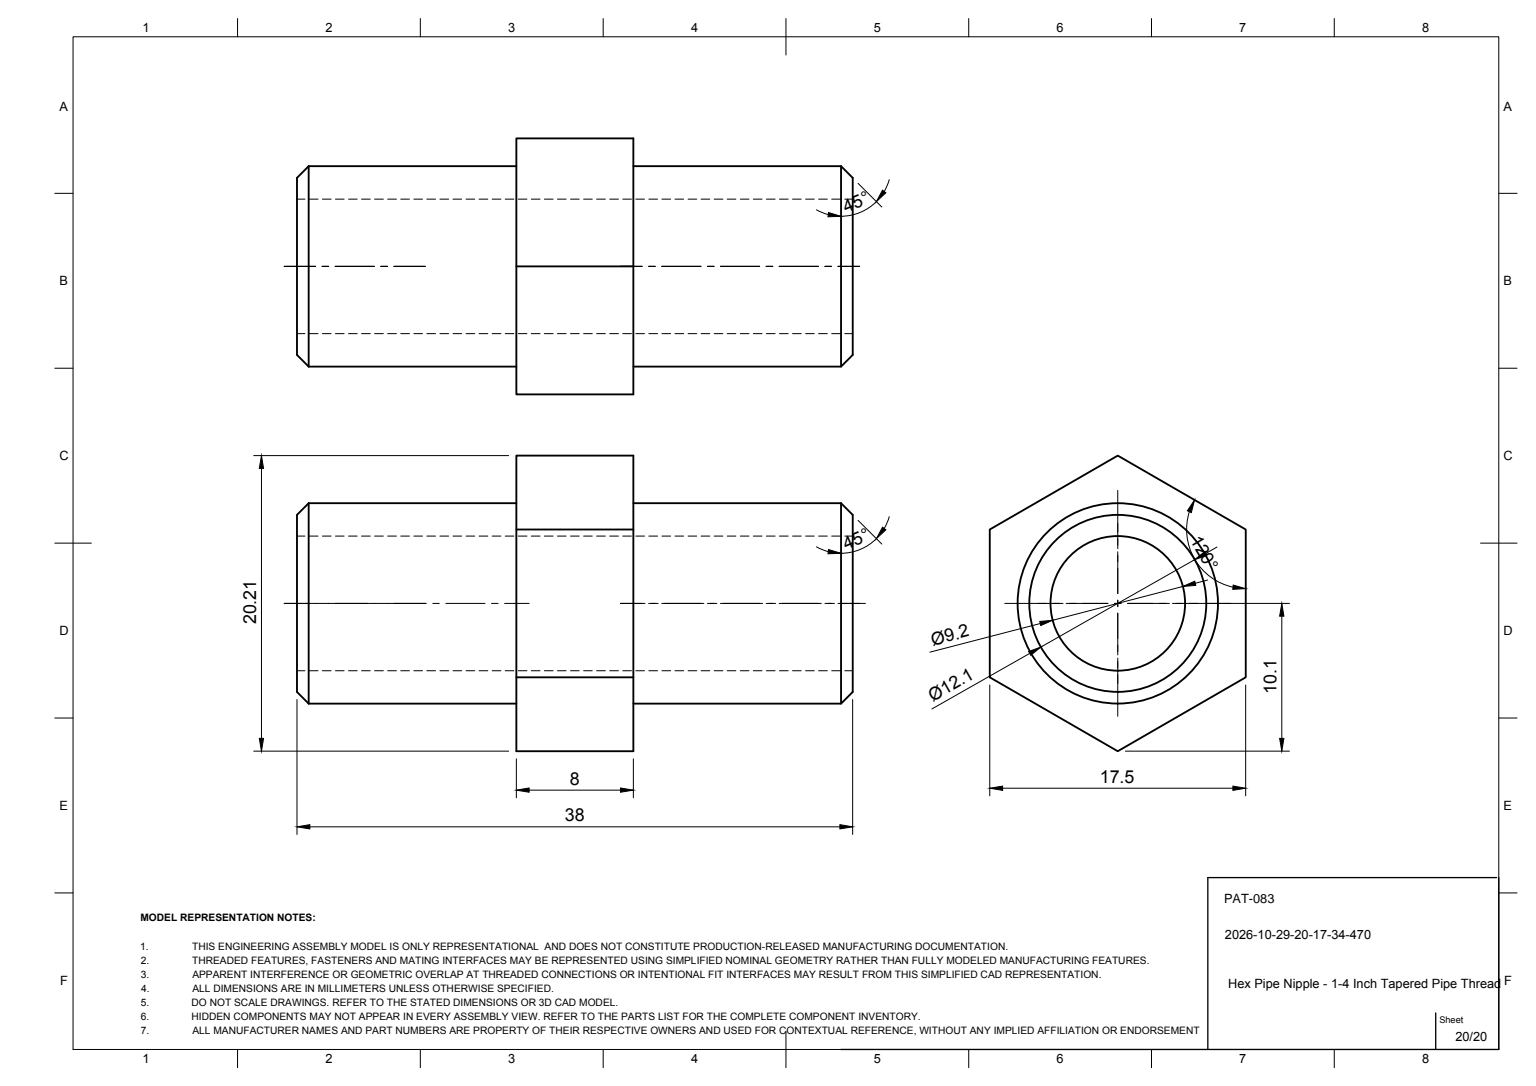
ISO-10303-21;
HEADER;
/* Generated by software containing ST-Developer
 * from STEP Tools, Inc. (www.steptools.com) 
 */

FILE_DESCRIPTION(
/* description */ ('PAT-083'),
/* implementation_level */ '2;1');

FILE_NAME(
/* name */ 'Hex Pipe Nipple - 1-4 Inch Tapered Pipe Thread.step',
/* time_stamp */ '2026-10-29T20:18:00-07:00',
/* author */ (''),
/* organization */ (''),
/* preprocessor_version */ 'ST-DEVELOPER v20.2',
/* originating_system */ 'Autodesk Translation Framework v15.17.0.0',
/* authorisation */ '');

FILE_SCHEMA (('AUTOMOTIVE_DESIGN { 1 0 10303 214 3 1 1 }'));
ENDSEC;

DATA;
#10=MECHANICAL_DESIGN_GEOMETRIC_PRESENTATION_REPRESENTATION('',(#248),#8428);
#153=CONICAL_SURFACE('',#4329,0.645,0.785398163397448);
#154=CONICAL_SURFACE('',#4332,0.645,0.785398163397448);
#200=SHAPE_REPRESENTATION_RELATIONSHIP('SRR','None',#8534,#224);
#224=ADVANCED_BREP_SHAPE_REPRESENTATION('',(#271),#8423);
#248=STYLED_ITEM('',(#8698),#271);
#271=MANIFOLD_SOLID_BREP('Body1',#3695);
#346=FACE_BOUND('',#974,.T.);
#347=FACE_BOUND('',#976,.T.);
#348=FACE_BOUND('',#985,.T.);
#349=FACE_BOUND('',#990,.T.);
#455=PLANE('',#4314);
#456=PLANE('',#4316);
#457=PLANE('',#4318);
#458=PLANE('',#4319);
#459=PLANE('',#4320);
#460=PLANE('',#4321);
#461=PLANE('',#4322);
#462=PLANE('',#4323);
#463=PLANE('',#4326);
#464=PLANE('',#4334);
#669=FACE_OUTER_BOUND('',#973,.T.);
#670=FACE_OUTER_BOUND('',#975,.T.);
#671=FACE_OUTER_BOUND('',#977,.T.);
#672=FACE_OUTER_BOUND('',#978,.T.);
#673=FACE_OUTER_BOUND('',#979,.T.);
#674=FACE_OUTER_BOUND('',#980,.T.);
#675=FACE_OUTER_BOUND('',#981,.T.);
#676=FACE_OUTER_BOUND('',#982,.T.);
#677=FACE_OUTER_BOUND('',#983,.T.);
#678=FACE_OUTER_BOUND('',#984,.T.);
#679=FACE_OUTER_BOUND('',#986,.T.);
#680=FACE_OUTER_BOUND('',#987,.T.);
#681=FACE_OUTER_BOUND('',#988,.T.);
#682=FACE_OUTER_BOUND('',#989,.T.);
#683=FACE_OUTER_BOUND('',#991,.T.);
#973=EDGE_LOOP('',(#3126,#3127,#3128,#3129,#3130,#3131));
#974=EDGE_LOOP('',(#3132));
#975=EDGE_LOOP('',(#3133,#3134,#3135,#3136,#3137,#3138));
#976=EDGE_LOOP('',(#3139));
#977=EDGE_LOOP('',(#3140,#3141,#3142,#3143));
#978=EDGE_LOOP('',(#3144,#3145,#3146,#3147));
#979=EDGE_LOOP('',(#3148,#3149,#3150,#3151));
#980=EDGE_LOOP('',(#3152,#3153,#3154,#3155));
#981=EDGE_LOOP('',(#3156,#3157,#3158,#3159));
#982=EDGE_LOOP('',(#3160,#3161,#3162,#3163));
#983=EDGE_LOOP('',(#3164,#3165,#3166,#3167));
#984=EDGE_LOOP('',(#3168));
#985=EDGE_LOOP('',(#3169));
#986=EDGE_LOOP('',(#3170,#3171,#3172,#3173));
#987=EDGE_LOOP('',(#3174,#3175,#3176,#3177));
#988=EDGE_LOOP('',(#3178,#3179,#3180,#3181));
#989=EDGE_LOOP('',(#3182));
#990=EDGE_LOOP('',(#3183));
#991=EDGE_LOOP('',(#3184,#3185,#3186,#3187));
#1207=LINE('',#8067,#1451);
#1208=LINE('',#8069,#1452);
#1209=LINE('',#8071,#1453);
#1210=LINE('',#8073,#1454);
#1211=LINE('',#8075,#1455);
#1212=LINE('',#8076,#1456);
#1213=LINE('',#8082,#1457);
#1214=LINE('',#8084,#1458);
#1215=LINE('',#8086,#1459);
#1216=LINE('',#8088,#1460);
#1217=LINE('',#8090,#1461);
#1218=LINE('',#8091,#1462);
#1219=LINE('',#8095,#1463);
#1220=LINE('',#8096,#1464);
#1221=LINE('',#8098,#1465);
#1222=LINE('',#8100,#1466);
#1223=LINE('',#8102,#1467);
#1224=LINE('',#8104,#1468);
#1225=LINE('',#8108,#1469);
#1226=LINE('',#8116,#1470);
#1227=LINE('',#8120,#1471);
#1228=LINE('',#8124,#1472);
#1229=LINE('',#8129,#1473);
#1451=VECTOR('',#5299,1.);
#1452=VECTOR('',#5300,1.);
#1453=VECTOR('',#5301,1.);
#1454=VECTOR('',#5302,1.);
#1455=VECTOR('',#5303,1.);
#1456=VECTOR('',#5304,1.);
#1457=VECTOR('',#5309,1.);
#1458=VECTOR('',#5310,1.);
#1459=VECTOR('',#5311,1.);
#1460=VECTOR('',#5312,1.);
#1461=VECTOR('',#5313,1.);
#1462=VECTOR('',#5314,1.);
#1463=VECTOR('',#5319,1.);
#1464=VECTOR('',#5320,1.);
#1465=VECTOR('',#5323,1.);
#1466=VECTOR('',#5326,1.);
#1467=VECTOR('',#5329,1.);
#1468=VECTOR('',#5332,1.);
#1469=VECTOR('',#5337,0.685);
#1470=VECTOR('',#5348,0.645);
#1471=VECTOR('',#5353,0.685);
#1472=VECTOR('',#5358,0.645);
#1473=VECTOR('',#5365,0.46);
#1685=CIRCLE('',#4315,0.685);
#1686=CIRCLE('',#4317,0.685);
#1687=CIRCLE('',#4325,0.685);
#1688=CIRCLE('',#4327,0.605);
#1689=CIRCLE('',#4328,0.46);
#1690=CIRCLE('',#4331,0.685);
#1691=CIRCLE('',#4333,0.605);
#1692=CIRCLE('',#4335,0.46);
#1929=VERTEX_POINT('',#8065);
#1930=VERTEX_POINT('',#8066);
#1931=VERTEX_POINT('',#8068);
#1932=VERTEX_POINT('',#8070);
#1933=VERTEX_POINT('',#8072);
#1934=VERTEX_POINT('',#8074);
#1935=VERTEX_POINT('',#8077);
#1936=VERTEX_POINT('',#8080);
#1937=VERTEX_POINT('',#8081);
#1938=VERTEX_POINT('',#8083);
#1939=VERTEX_POINT('',#8085);
#1940=VERTEX_POINT('',#8087);
#1941=VERTEX_POINT('',#8089);
#1942=VERTEX_POINT('',#8092);
#1943=VERTEX_POINT('',#8107);
#1944=VERTEX_POINT('',#8111);
#1945=VERTEX_POINT('',#8113);
#1946=VERTEX_POINT('',#8118);
#1947=VERTEX_POINT('',#8122);
#1948=VERTEX_POINT('',#8126);
#2339=EDGE_CURVE('',#1929,#1930,#1207,.T.);
#2340=EDGE_CURVE('',#1930,#1931,#1208,.T.);
#2341=EDGE_CURVE('',#1931,#1932,#1209,.T.);
#2342=EDGE_CURVE('',#1932,#1933,#1210,.T.);
#2343=EDGE_CURVE('',#1933,#1934,#1211,.T.);
#2344=EDGE_CURVE('',#1934,#1929,#1212,.T.);
#2345=EDGE_CURVE('',#1935,#1935,#1685,.T.);
#2346=EDGE_CURVE('',#1936,#1937,#1213,.T.);
#2347=EDGE_CURVE('',#1937,#1938,#1214,.T.);
#2348=EDGE_CURVE('',#1938,#1939,#1215,.T.);
#2349=EDGE_CURVE('',#1939,#1940,#1216,.T.);
#2350=EDGE_CURVE('',#1940,#1941,#1217,.T.);
#2351=EDGE_CURVE('',#1941,#1936,#1218,.T.);
#2352=EDGE_CURVE('',#1942,#1942,#1686,.T.);
#2353=EDGE_CURVE('',#1936,#1930,#1219,.T.);
#2354=EDGE_CURVE('',#1931,#1941,#1220,.T.);
#2355=EDGE_CURVE('',#1932,#1940,#1221,.T.);
#2356=EDGE_CURVE('',#1933,#1939,#1222,.T.);
#2357=EDGE_CURVE('',#1934,#1938,#1223,.T.);
#2358=EDGE_CURVE('',#1929,#1937,#1224,.T.);
#2359=EDGE_CURVE('',#1942,#1943,#1225,.T.);
#2360=EDGE_CURVE('',#1943,#1943,#1687,.T.);
#2361=EDGE_CURVE('',#1944,#1944,#1688,.T.);
#2362=EDGE_CURVE('',#1945,#1945,#1689,.T.);
#2363=EDGE_CURVE('',#1943,#1944,#1226,.T.);
#2364=EDGE_CURVE('',#1946,#1946,#1690,.T.);
#2365=EDGE_CURVE('',#1946,#1935,#1227,.T.);
#2366=EDGE_CURVE('',#1947,#1947,#1691,.T.);
#2367=EDGE_CURVE('',#1947,#1946,#1228,.T.);
#2368=EDGE_CURVE('',#1948,#1948,#1692,.T.);
#2369=EDGE_CURVE('',#1948,#1945,#1229,.T.);
#3126=ORIENTED_EDGE('',*,*,#2339,.T.);
#3127=ORIENTED_EDGE('',*,*,#2340,.T.);
#3128=ORIENTED_EDGE('',*,*,#2341,.T.);
#3129=ORIENTED_EDGE('',*,*,#2342,.T.);
#3130=ORIENTED_EDGE('',*,*,#2343,.T.);
#3131=ORIENTED_EDGE('',*,*,#2344,.T.);
#3132=ORIENTED_EDGE('',*,*,#2345,.F.);
#3133=ORIENTED_EDGE('',*,*,#2346,.T.);
#3134=ORIENTED_EDGE('',*,*,#2347,.T.);
#3135=ORIENTED_EDGE('',*,*,#2348,.T.);
#3136=ORIENTED_EDGE('',*,*,#2349,.T.);
#3137=ORIENTED_EDGE('',*,*,#2350,.T.);
#3138=ORIENTED_EDGE('',*,*,#2351,.T.);
#3139=ORIENTED_EDGE('',*,*,#2352,.F.);
#3140=ORIENTED_EDGE('',*,*,#2353,.F.);
#3141=ORIENTED_EDGE('',*,*,#2351,.F.);
#3142=ORIENTED_EDGE('',*,*,#2354,.F.);
#3143=ORIENTED_EDGE('',*,*,#2340,.F.);
#3144=ORIENTED_EDGE('',*,*,#2354,.T.);
#3145=ORIENTED_EDGE('',*,*,#2350,.F.);
#3146=ORIENTED_EDGE('',*,*,#2355,.F.);
#3147=ORIENTED_EDGE('',*,*,#2341,.F.);
#3148=ORIENTED_EDGE('',*,*,#2355,.T.);
#3149=ORIENTED_EDGE('',*,*,#2349,.F.);
#3150=ORIENTED_EDGE('',*,*,#2356,.F.);
#3151=ORIENTED_EDGE('',*,*,#2342,.F.);
#3152=ORIENTED_EDGE('',*,*,#2356,.T.);
#3153=ORIENTED_EDGE('',*,*,#2348,.F.);
#3154=ORIENTED_EDGE('',*,*,#2357,.F.);
#3155=ORIENTED_EDGE('',*,*,#2343,.F.);
#3156=ORIENTED_EDGE('',*,*,#2357,.T.);
#3157=ORIENTED_EDGE('',*,*,#2347,.F.);
#3158=ORIENTED_EDGE('',*,*,#2358,.F.);
#3159=ORIENTED_EDGE('',*,*,#2344,.F.);
#3160=ORIENTED_EDGE('',*,*,#2358,.T.);
#3161=ORIENTED_EDGE('',*,*,#2346,.F.);
#3162=ORIENTED_EDGE('',*,*,#2353,.T.);
#3163=ORIENTED_EDGE('',*,*,#2339,.F.);
#3164=ORIENTED_EDGE('',*,*,#2352,.T.);
#3165=ORIENTED_EDGE('',*,*,#2359,.T.);
#3166=ORIENTED_EDGE('',*,*,#2360,.T.);
#3167=ORIENTED_EDGE('',*,*,#2359,.F.);
#3168=ORIENTED_EDGE('',*,*,#2361,.F.);
#3169=ORIENTED_EDGE('',*,*,#2362,.T.);
#3170=ORIENTED_EDGE('',*,*,#2360,.F.);
#3171=ORIENTED_EDGE('',*,*,#2363,.T.);
#3172=ORIENTED_EDGE('',*,*,#2361,.T.);
#3173=ORIENTED_EDGE('',*,*,#2363,.F.);
#3174=ORIENTED_EDGE('',*,*,#2364,.F.);
#3175=ORIENTED_EDGE('',*,*,#2365,.T.);
#3176=ORIENTED_EDGE('',*,*,#2345,.T.);
#3177=ORIENTED_EDGE('',*,*,#2365,.F.);
#3178=ORIENTED_EDGE('',*,*,#2366,.F.);
#3179=ORIENTED_EDGE('',*,*,#2367,.T.);
#3180=ORIENTED_EDGE('',*,*,#2364,.T.);
#3181=ORIENTED_EDGE('',*,*,#2367,.F.);
#3182=ORIENTED_EDGE('',*,*,#2366,.T.);
#3183=ORIENTED_EDGE('',*,*,#2368,.F.);
#3184=ORIENTED_EDGE('',*,*,#2368,.T.);
#3185=ORIENTED_EDGE('',*,*,#2369,.T.);
#3186=ORIENTED_EDGE('',*,*,#2362,.F.);
#3187=ORIENTED_EDGE('',*,*,#2369,.F.);
#3433=CYLINDRICAL_SURFACE('',#4324,0.685);
#3434=CYLINDRICAL_SURFACE('',#4330,0.685);
#3435=CYLINDRICAL_SURFACE('',#4336,0.46);
#3616=ADVANCED_FACE('',(#669,#346),#455,.F.);
#3617=ADVANCED_FACE('',(#670,#347),#456,.T.);
#3618=ADVANCED_FACE('',(#671),#457,.T.);
#3619=ADVANCED_FACE('',(#672),#458,.T.);
#3620=ADVANCED_FACE('',(#673),#459,.T.);
#3621=ADVANCED_FACE('',(#674),#460,.T.);
#3622=ADVANCED_FACE('',(#675),#461,.T.);
#3623=ADVANCED_FACE('',(#676),#462,.T.);
#3624=ADVANCED_FACE('',(#677),#3433,.T.);
#3625=ADVANCED_FACE('',(#678,#348),#463,.T.);
#3626=ADVANCED_FACE('',(#679),#153,.T.);
#3627=ADVANCED_FACE('',(#680),#3434,.T.);
#3628=ADVANCED_FACE('',(#681),#154,.T.);
#3629=ADVANCED_FACE('',(#682,#349),#464,.T.);
#3630=ADVANCED_FACE('',(#683),#3435,.F.);
#3695=CLOSED_SHELL('',(#3616,#3617,#3618,#3619,#3620,#3621,#3622,#3623,
#3624,#3625,#3626,#3627,#3628,#3629,#3630));
#4313=AXIS2_PLACEMENT_3D('',#8063,#5295,#5296);
#4314=AXIS2_PLACEMENT_3D('',#8064,#5297,#5298);
#4315=AXIS2_PLACEMENT_3D('',#8078,#5305,#5306);
#4316=AXIS2_PLACEMENT_3D('',#8079,#5307,#5308);
#4317=AXIS2_PLACEMENT_3D('',#8093,#5315,#5316);
#4318=AXIS2_PLACEMENT_3D('',#8094,#5317,#5318);
#4319=AXIS2_PLACEMENT_3D('',#8097,#5321,#5322);
#4320=AXIS2_PLACEMENT_3D('',#8099,#5324,#5325);
#4321=AXIS2_PLACEMENT_3D('',#8101,#5327,#5328);
#4322=AXIS2_PLACEMENT_3D('',#8103,#5330,#5331);
#4323=AXIS2_PLACEMENT_3D('',#8105,#5333,#5334);
#4324=AXIS2_PLACEMENT_3D('',#8106,#5335,#5336);
#4325=AXIS2_PLACEMENT_3D('',#8109,#5338,#5339);
#4326=AXIS2_PLACEMENT_3D('',#8110,#5340,#5341);
#4327=AXIS2_PLACEMENT_3D('',#8112,#5342,#5343);
#4328=AXIS2_PLACEMENT_3D('',#8114,#5344,#5345);
#4329=AXIS2_PLACEMENT_3D('',#8115,#5346,#5347);
#4330=AXIS2_PLACEMENT_3D('',#8117,#5349,#5350);
#4331=AXIS2_PLACEMENT_3D('',#8119,#5351,#5352);
#4332=AXIS2_PLACEMENT_3D('',#8121,#5354,#5355);
#4333=AXIS2_PLACEMENT_3D('',#8123,#5356,#5357);
#4334=AXIS2_PLACEMENT_3D('',#8125,#5359,#5360);
#4335=AXIS2_PLACEMENT_3D('',#8127,#5361,#5362);
#4336=AXIS2_PLACEMENT_3D('',#8128,#5363,#5364);
#5295=DIRECTION('axis',(0.,0.,1.));
#5296=DIRECTION('refdir',(1.,0.,0.));
#5297=DIRECTION('center_axis',(0.,1.,0.));
#5298=DIRECTION('ref_axis',(1.,0.,0.));
#5299=DIRECTION('',(-0.5,0.,0.866025403784439));
#5300=DIRECTION('',(-1.,0.,-3.29650746237182E-16));
#5301=DIRECTION('',(-0.5,0.,-0.866025403784439));
#5302=DIRECTION('',(0.5,0.,-0.866025403784438));
#5303=DIRECTION('',(1.,0.,0.));
#5304=DIRECTION('',(0.5,0.,0.866025403784439));
#5305=DIRECTION('center_axis',(0.,-1.,0.));
#5306=DIRECTION('ref_axis',(1.,0.,0.));
#5307=DIRECTION('center_axis',(0.,1.,0.));
#5308=DIRECTION('ref_axis',(1.,0.,0.));
#5309=DIRECTION('',(0.5,0.,-0.866025403784439));
#5310=DIRECTION('',(-0.5,0.,-0.866025403784439));
#5311=DIRECTION('',(-1.,0.,0.));
#5312=DIRECTION('',(-0.5,0.,0.866025403784438));
#5313=DIRECTION('',(0.5,0.,0.866025403784439));
#5314=DIRECTION('',(1.,0.,3.29650746237182E-16));
#5315=DIRECTION('center_axis',(0.,1.,0.));
#5316=DIRECTION('ref_axis',(1.,0.,0.));
#5317=DIRECTION('center_axis',(-3.29650746237182E-16,0.,1.));
#5318=DIRECTION('ref_axis',(1.,0.,3.29650746237182E-16));
#5319=DIRECTION('',(0.,-1.,0.));
#5320=DIRECTION('',(0.,1.,0.));
#5321=DIRECTION('center_axis',(-0.866025403784439,0.,0.5));
#5322=DIRECTION('ref_axis',(0.5,0.,0.866025403784439));
#5323=DIRECTION('',(0.,1.,0.));
#5324=DIRECTION('center_axis',(-0.866025403784439,0.,-0.5));
#5325=DIRECTION('ref_axis',(-0.5,0.,0.866025403784439));
#5326=DIRECTION('',(0.,1.,0.));
#5327=DIRECTION('center_axis',(0.,0.,-1.));
#5328=DIRECTION('ref_axis',(-1.,0.,0.));
#5329=DIRECTION('',(0.,1.,0.));
#5330=DIRECTION('center_axis',(0.866025403784439,0.,-0.5));
#5331=DIRECTION('ref_axis',(-0.5,0.,-0.866025403784439));
#5332=DIRECTION('',(0.,1.,0.));
#5333=DIRECTION('center_axis',(0.866025403784439,0.,0.5));
#5334=DIRECTION('ref_axis',(0.5,0.,-0.866025403784439));
#5335=DIRECTION('center_axis',(0.,-1.,0.));
#5336=DIRECTION('ref_axis',(1.,0.,0.));
#5337=DIRECTION('',(0.,1.,0.));
#5338=DIRECTION('center_axis',(0.,-1.,0.));
#5339=DIRECTION('ref_axis',(1.,0.,0.));
#5340=DIRECTION('center_axis',(0.,1.,0.));
#5341=DIRECTION('ref_axis',(0.,0.,1.));
#5342=DIRECTION('center_axis',(0.,-1.,0.));
#5343=DIRECTION('ref_axis',(1.,0.,0.));
#5344=DIRECTION('center_axis',(0.,-1.,0.));
#5345=DIRECTION('ref_axis',(1.,0.,0.));
#5346=DIRECTION('center_axis',(0.,-1.,0.));
#5347=DIRECTION('ref_axis',(1.,0.,0.));
#5348=DIRECTION('',(0.707106781186547,0.707106781186548,8.65956056235493E-17));
#5349=DIRECTION('center_axis',(0.,-1.,0.));
#5350=DIRECTION('ref_axis',(1.,0.,0.));
#5351=DIRECTION('center_axis',(0.,-1.,0.));
#5352=DIRECTION('ref_axis',(1.,0.,0.));
#5353=DIRECTION('',(0.,1.,0.));
#5354=DIRECTION('center_axis',(0.,1.,0.));
#5355=DIRECTION('ref_axis',(1.,0.,0.));
#5356=DIRECTION('center_axis',(0.,-1.,0.));
#5357=DIRECTION('ref_axis',(1.,0.,0.));
#5358=DIRECTION('',(-0.707106781186547,0.707106781186548,-8.65956056235493E-17));
#5359=DIRECTION('center_axis',(0.,-1.,0.));
#5360=DIRECTION('ref_axis',(0.,0.,-1.));
#5361=DIRECTION('center_axis',(0.,-1.,0.));
#5362=DIRECTION('ref_axis',(1.,0.,0.));
#5363=DIRECTION('center_axis',(0.,-1.,0.));
#5364=DIRECTION('ref_axis',(1.,0.,0.));
#5365=DIRECTION('',(0.,1.,0.));
#8063=CARTESIAN_POINT('',(0.,0.,0.));
#8064=CARTESIAN_POINT('Origin',(0.,-0.4,0.));
#8065=CARTESIAN_POINT('',(1.01036297108185,-0.4,0.));
#8066=CARTESIAN_POINT('',(0.505181485540923,-0.4,0.875));
#8067=CARTESIAN_POINT('',(0.505181485540923,-0.4,0.875));
#8068=CARTESIAN_POINT('',(-0.505181485540923,-0.4,0.875));
#8069=CARTESIAN_POINT('',(-0.505181485540923,-0.4,0.875));
#8070=CARTESIAN_POINT('',(-1.01036297108185,-0.4,-1.23733777851239E-16));
#8071=CARTESIAN_POINT('',(-1.01036297108185,-0.4,-1.23733777851239E-16));
#8072=CARTESIAN_POINT('',(-0.505181485540922,-0.4,-0.875));
#8073=CARTESIAN_POINT('',(-0.505181485540922,-0.4,-0.875));
#8074=CARTESIAN_POINT('',(0.505181485540923,-0.4,-0.875));
#8075=CARTESIAN_POINT('',(0.505181485540923,-0.4,-0.875));
#8076=CARTESIAN_POINT('',(1.01036297108185,-0.4,0.));
#8077=CARTESIAN_POINT('',(-0.685,-0.4,-8.38883057415937E-17));
#8078=CARTESIAN_POINT('Origin',(0.,-0.4,0.));
#8079=CARTESIAN_POINT('Origin',(0.,0.4,0.));
#8080=CARTESIAN_POINT('',(0.505181485540923,0.4,0.875));
#8081=CARTESIAN_POINT('',(1.01036297108185,0.4,0.));
#8082=CARTESIAN_POINT('',(0.505181485540923,0.4,0.875));
#8083=CARTESIAN_POINT('',(0.505181485540923,0.4,-0.875));
#8084=CARTESIAN_POINT('',(1.01036297108185,0.4,0.));
#8085=CARTESIAN_POINT('',(-0.505181485540922,0.4,-0.875));
#8086=CARTESIAN_POINT('',(0.505181485540923,0.4,-0.875));
#8087=CARTESIAN_POINT('',(-1.01036297108185,0.4,-1.23733777851239E-16));
#8088=CARTESIAN_POINT('',(-0.505181485540922,0.4,-0.875));
#8089=CARTESIAN_POINT('',(-0.505181485540923,0.4,0.875));
#8090=CARTESIAN_POINT('',(-1.01036297108185,0.4,-1.23733777851239E-16));
#8091=CARTESIAN_POINT('',(-0.505181485540923,0.4,0.875));
#8092=CARTESIAN_POINT('',(-0.685,0.4,8.38883057415937E-17));
#8093=CARTESIAN_POINT('Origin',(0.,0.4,0.));
#8094=CARTESIAN_POINT('Origin',(-0.505181485540923,0.,0.875));
#8095=CARTESIAN_POINT('',(0.505181485540923,0.,0.875));
#8096=CARTESIAN_POINT('',(-0.505181485540923,0.,0.875));
#8097=CARTESIAN_POINT('Origin',(-1.01036297108185,0.,-1.23733777851239E-16));
#8098=CARTESIAN_POINT('',(-1.01036297108185,0.,-1.23733777851239E-16));
#8099=CARTESIAN_POINT('Origin',(-0.505181485540922,0.,-0.875));
#8100=CARTESIAN_POINT('',(-0.505181485540922,0.,-0.875));
#8101=CARTESIAN_POINT('Origin',(0.505181485540923,0.,-0.875));
#8102=CARTESIAN_POINT('',(0.505181485540923,0.,-0.875));
#8103=CARTESIAN_POINT('Origin',(1.01036297108185,0.,0.));
#8104=CARTESIAN_POINT('',(1.01036297108185,0.,0.));
#8105=CARTESIAN_POINT('Origin',(0.505181485540923,0.,0.875));
#8106=CARTESIAN_POINT('Origin',(0.,0.,0.));
#8107=CARTESIAN_POINT('',(-0.685,1.82,-8.38883057415937E-17));
#8108=CARTESIAN_POINT('',(-0.685,0.,-8.38883057415937E-17));
#8109=CARTESIAN_POINT('Origin',(0.,1.82,0.));
#8110=CARTESIAN_POINT('Origin',(0.605,1.9,0.));
#8111=CARTESIAN_POINT('',(-0.605,1.9,-7.40911313484149E-17));
#8112=CARTESIAN_POINT('Origin',(0.,1.9,0.));
#8113=CARTESIAN_POINT('',(-0.46,1.9,-5.63337527607782E-17));
#8114=CARTESIAN_POINT('Origin',(0.,1.9,0.));
#8115=CARTESIAN_POINT('Origin',(0.,1.86,0.));
#8116=CARTESIAN_POINT('',(-0.645,1.86,-7.89897185450043E-17));
#8117=CARTESIAN_POINT('Origin',(0.,0.,0.));
#8118=CARTESIAN_POINT('',(-0.685,-1.82,-8.38883057415937E-17));
#8119=CARTESIAN_POINT('Origin',(0.,-1.82,0.));
#8120=CARTESIAN_POINT('',(-0.685,0.,-8.38883057415937E-17));
#8121=CARTESIAN_POINT('Origin',(0.,-1.86,0.));
#8122=CARTESIAN_POINT('',(-0.605,-1.9,-7.40911313484149E-17));
#8123=CARTESIAN_POINT('Origin',(0.,-1.9,0.));
#8124=CARTESIAN_POINT('',(-0.645,-1.86,-7.89897185450043E-17));
#8125=CARTESIAN_POINT('Origin',(0.46,-1.9,0.));
#8126=CARTESIAN_POINT('',(-0.46,-1.9,-5.63337527607782E-17));
#8127=CARTESIAN_POINT('Origin',(0.,-1.9,0.));
#8128=CARTESIAN_POINT('Origin',(0.,0.,0.));
#8129=CARTESIAN_POINT('',(-0.46,0.,-5.63337527607782E-17));
#8397=UNCERTAINTY_MEASURE_WITH_UNIT(LENGTH_MEASURE(0.001),#8429,
'DISTANCE_ACCURACY_VALUE',
'Maximum model space distance between geometric entities at asserted c
onnectivities');
#8402=UNCERTAINTY_MEASURE_WITH_UNIT(LENGTH_MEASURE(0.001),#8429,
'DISTANCE_ACCURACY_VALUE',
'Maximum model space distance between geometric entities at asserted c
onnectivities');
#8423=(
GEOMETRIC_REPRESENTATION_CONTEXT(3)
GLOBAL_UNCERTAINTY_ASSIGNED_CONTEXT((#8397))
GLOBAL_UNIT_ASSIGNED_CONTEXT((#8429,#8431,#8432))
REPRESENTATION_CONTEXT('','3D')
);
#8428=(
GEOMETRIC_REPRESENTATION_CONTEXT(3)
GLOBAL_UNCERTAINTY_ASSIGNED_CONTEXT((#8402))
GLOBAL_UNIT_ASSIGNED_CONTEXT((#8429,#8431,#8432))
REPRESENTATION_CONTEXT('','3D')
);
#8429=(
LENGTH_UNIT()
NAMED_UNIT(*)
SI_UNIT(.CENTI.,.METRE.)
);
#8431=(
NAMED_UNIT(*)
PLANE_ANGLE_UNIT()
SI_UNIT($,.RADIAN.)
);
#8432=(
NAMED_UNIT(*)
SI_UNIT($,.STERADIAN.)
SOLID_ANGLE_UNIT()
);
#8453=SHAPE_DEFINITION_REPRESENTATION(#8478,#8534);
#8478=PRODUCT_DEFINITION_SHAPE('',$,#8560);
#8534=SHAPE_REPRESENTATION('',(#4313),#8423);
#8539=PRODUCT_DEFINITION_CONTEXT('part definition',#8616,'design');
#8560=PRODUCT_DEFINITION('Hex Pipe Nipple - 1-4 Inch Tapered Pipe Thread',
'Hex Pipe Nipple - 1-4 Inch Tapered Pipe Thread',#8585,#8539);
#8585=PRODUCT_DEFINITION_FORMATION('',$,#8638);
#8616=APPLICATION_CONTEXT(
'Core Data for Automotive Mechanical Design Process');
#8617=PRODUCT_CONTEXT('part definition',#8616,'mechanical');
#8638=PRODUCT('Hex Pipe Nipple - 1-4 Inch Tapered Pipe Thread',
'Hex Pipe Nipple - 1-4 Inch Tapered Pipe Thread',
'Hex Pipe Nipple - 1-4 Inch Tapered Pipe Thread',(#8617));
#8692=COLOUR_RGB('Sky Blue',0.24,0.69,0.87);
#8693=FILL_AREA_STYLE_COLOUR('',#8692);
#8694=FILL_AREA_STYLE('',(#8693));
#8695=SURFACE_STYLE_FILL_AREA(#8694);
#8696=SURFACE_SIDE_STYLE('',(#8695));
#8697=SURFACE_STYLE_USAGE(.BOTH.,#8696);
#8698=PRESENTATION_STYLE_ASSIGNMENT((#8697));
ENDSEC;
END-ISO-10303-21;
